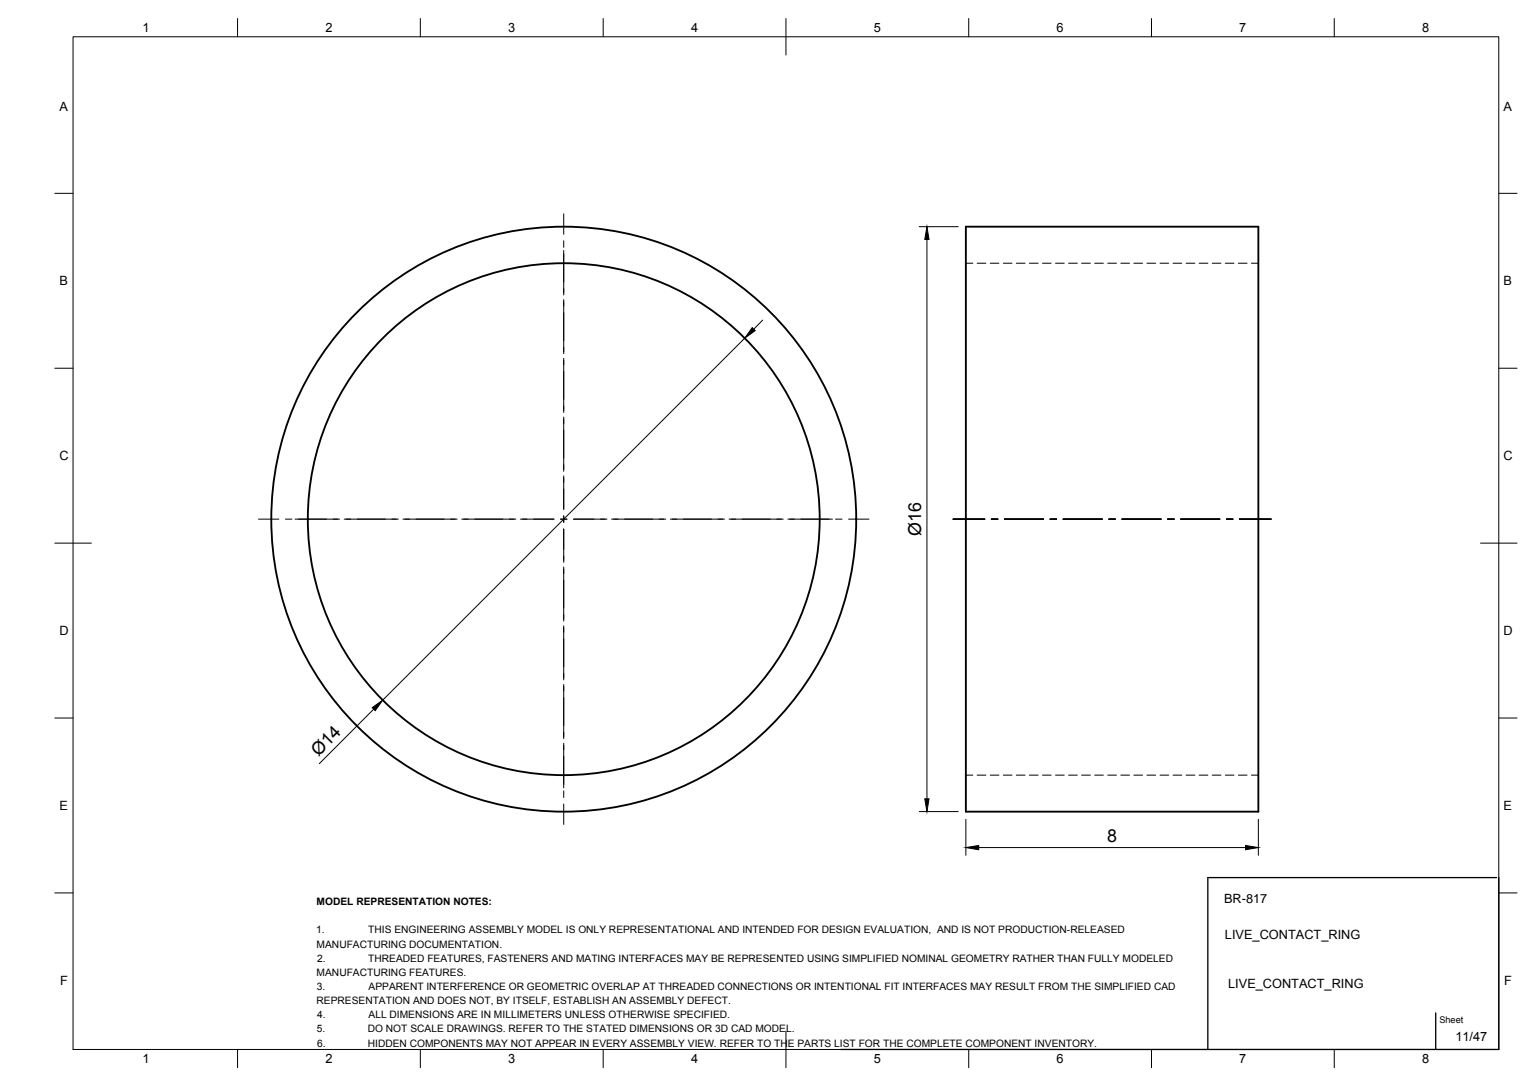
ISO-10303-21;
HEADER;
FILE_DESCRIPTION((''),'2;1');
FILE_NAME('LIVE_CONTACT_RING.step','2026-10-01T22:07:29-07:00',(''),(''),'','','');
FILE_SCHEMA (('AUTOMOTIVE_DESIGN { 1 0 10303 214 3 1 1 }'));
ENDSEC;
DATA;
#10=MECHANICAL_DESIGN_GEOMETRIC_PRESENTATION_REPRESENTATION('',(#547),#15484);
#477=SHAPE_REPRESENTATION_RELATIONSHIP('SRR','None',#15625,#512) ;
#512=ADVANCED_BREP_SHAPE_REPRESENTATION('',(#589),#15449) ;
#547=STYLED_ITEM('',(#15834),#589) ;
#589=MANIFOLD_SOLID_BREP('LIVE_CONTACT_RING',#8256) ;
#654=CYLINDRICAL_SURFACE('',#8850,0.7) ;
#655=CYLINDRICAL_SURFACE('',#8853,0.8) ;
#847=FACE_BOUND('',#2007,.T.) ;
#848=FACE_BOUND('',#2009,.T.) ;
#941=CIRCLE('',#8851,0.7) ;
#942=CIRCLE('',#8852,0.7) ;
#943=CIRCLE('',#8854,0.8) ;
#944=CIRCLE('',#8855,0.8) ;
#1467=FACE_OUTER_BOUND('',#2004,.T.) ;
#1468=FACE_OUTER_BOUND('',#2005,.T.) ;
#1469=FACE_OUTER_BOUND('',#2006,.T.) ;
#1470=FACE_OUTER_BOUND('',#2008,.T.) ;
#2004=EDGE_LOOP('',(#5723,#5724,#5725,#5726)) ;
#2005=EDGE_LOOP('',(#5727,#5728,#5729,#5730)) ;
#2006=EDGE_LOOP('',(#5731)) ;
#2007=EDGE_LOOP('',(#5732)) ;
#2008=EDGE_LOOP('',(#5733)) ;
#2009=EDGE_LOOP('',(#5734)) ;
#2609=LINE('',#13376,#3083) ;
#2610=LINE('',#13382,#3084) ;
#3083=VECTOR('',#10434,0.7) ;
#3084=VECTOR('',#10441,0.8) ;
#3538=VERTEX_POINT('',#13373) ;
#3539=VERTEX_POINT('',#13375) ;
#3540=VERTEX_POINT('',#13379) ;
#3541=VERTEX_POINT('',#13381) ;
#4366=EDGE_CURVE('',#3538,#3538,#941,.T.) ;
#4367=EDGE_CURVE('',#3538,#3539,#2609,.T.) ;
#4368=EDGE_CURVE('',#3539,#3539,#942,.T.) ;
#4369=EDGE_CURVE('',#3540,#3540,#943,.T.) ;
#4370=EDGE_CURVE('',#3540,#3541,#2610,.T.) ;
#4371=EDGE_CURVE('',#3541,#3541,#944,.T.) ;
#5723=ORIENTED_EDGE('',*,*,#4366,.F.) ;
#5724=ORIENTED_EDGE('',*,*,#4367,.T.) ;
#5725=ORIENTED_EDGE('',*,*,#4368,.F.) ;
#5726=ORIENTED_EDGE('',*,*,#4367,.F.) ;
#5727=ORIENTED_EDGE('',*,*,#4369,.F.) ;
#5728=ORIENTED_EDGE('',*,*,#4370,.T.) ;
#5729=ORIENTED_EDGE('',*,*,#4371,.F.) ;
#5730=ORIENTED_EDGE('',*,*,#4370,.F.) ;
#5731=ORIENTED_EDGE('',*,*,#4371,.T.) ;
#5732=ORIENTED_EDGE('',*,*,#4366,.T.) ;
#5733=ORIENTED_EDGE('',*,*,#4369,.T.) ;
#5734=ORIENTED_EDGE('',*,*,#4368,.T.) ;
#7611=PLANE('',#8856) ;
#7612=PLANE('',#8857) ;
#7854=ADVANCED_FACE('',(#1467),#654,.F.) ;
#7855=ADVANCED_FACE('',(#1468),#655,.T.) ;
#7856=ADVANCED_FACE('',(#1469,#847),#7611,.T.) ;
#7857=ADVANCED_FACE('',(#1470,#848),#7612,.T.) ;
#8256=CLOSED_SHELL('',(#7854,#7855,#7856,#7857)) ;
#8849=AXIS2_PLACEMENT_3D('',#13371,#10428,#10429) ;
#8850=AXIS2_PLACEMENT_3D('',#13372,#10430,#10431) ;
#8851=AXIS2_PLACEMENT_3D('',#13374,#10432,#10433) ;
#8852=AXIS2_PLACEMENT_3D('',#13377,#10435,#10436) ;
#8853=AXIS2_PLACEMENT_3D('',#13378,#10437,#10438) ;
#8854=AXIS2_PLACEMENT_3D('',#13380,#10439,#10440) ;
#8855=AXIS2_PLACEMENT_3D('',#13383,#10442,#10443) ;
#8856=AXIS2_PLACEMENT_3D('',#13384,#10444,#10445) ;
#8857=AXIS2_PLACEMENT_3D('',#13385,#10446,#10447) ;
#10428=DIRECTION('axis',(0.,0.,1.)) ;
#10429=DIRECTION('refdir',(1.,0.,0.)) ;
#10430=DIRECTION('center_axis',(0.,0.,1.)) ;
#10431=DIRECTION('ref_axis',(1.,0.,0.)) ;
#10432=DIRECTION('center_axis',(0.,0.,1.)) ;
#10433=DIRECTION('ref_axis',(1.,0.,0.)) ;
#10434=DIRECTION('',(0.,0.,1.)) ;
#10435=DIRECTION('center_axis',(0.,0.,-1.)) ;
#10436=DIRECTION('ref_axis',(1.,0.,0.)) ;
#10437=DIRECTION('center_axis',(0.,0.,1.)) ;
#10438=DIRECTION('ref_axis',(1.,0.,0.)) ;
#10439=DIRECTION('center_axis',(0.,0.,1.)) ;
#10440=DIRECTION('ref_axis',(1.,0.,0.)) ;
#10441=DIRECTION('',(0.,0.,-1.)) ;
#10442=DIRECTION('center_axis',(0.,0.,-1.)) ;
#10443=DIRECTION('ref_axis',(1.,0.,0.)) ;
#10444=DIRECTION('center_axis',(0.,0.,-1.)) ;
#10445=DIRECTION('ref_axis',(-1.,0.,0.)) ;
#10446=DIRECTION('center_axis',(0.,0.,1.)) ;
#10447=DIRECTION('ref_axis',(1.,0.,0.)) ;
#13371=CARTESIAN_POINT('',(0.,0.,0.)) ;
#13372=CARTESIAN_POINT('Origin',(-1.,0.,-0.7)) ;
#13373=CARTESIAN_POINT('',(-1.7,-8.57252759403147E-17,-1.1)) ;
#13374=CARTESIAN_POINT('Origin',(-1.,0.,-1.1)) ;
#13375=CARTESIAN_POINT('',(-1.7,8.57252759403147E-17,-0.3)) ;
#13376=CARTESIAN_POINT('',(-1.7,-8.57252759403147E-17,-0.7)) ;
#13377=CARTESIAN_POINT('Origin',(-1.,0.,-0.3)) ;
#13378=CARTESIAN_POINT('Origin',(-1.,0.,-0.7)) ;
#13379=CARTESIAN_POINT('',(-1.8,-9.79717439317883E-17,-0.3)) ;
#13380=CARTESIAN_POINT('Origin',(-1.,0.,-0.3)) ;
#13381=CARTESIAN_POINT('',(-1.8,-9.79717439317883E-17,-1.1)) ;
#13382=CARTESIAN_POINT('',(-1.8,-9.79717439317883E-17,-0.7)) ;
#13383=CARTESIAN_POINT('Origin',(-1.,0.,-1.1)) ;
#13384=CARTESIAN_POINT('Origin',(-1.,0.,-1.1)) ;
#13385=CARTESIAN_POINT('Origin',(-1.,0.,-0.3)) ;
#15406=UNCERTAINTY_MEASURE_WITH_UNIT(LENGTH_MEASURE(0.001),#15485,
'DISTANCE_ACCURACY_VALUE',
'Maximum model space distance between geometric entities at asserted c
onnectivities') ;
#15441=UNCERTAINTY_MEASURE_WITH_UNIT(LENGTH_MEASURE(0.001),#15485,
'DISTANCE_ACCURACY_VALUE',
'Maximum model space distance between geometric entities at asserted c
onnectivities') ;
#15449=(
GEOMETRIC_REPRESENTATION_CONTEXT(3)
GLOBAL_UNCERTAINTY_ASSIGNED_CONTEXT((#15406))
GLOBAL_UNIT_ASSIGNED_CONTEXT((#15485,#15487,#15488))
REPRESENTATION_CONTEXT('','3D')
) ;
#15484=(
GEOMETRIC_REPRESENTATION_CONTEXT(3)
GLOBAL_UNCERTAINTY_ASSIGNED_CONTEXT((#15441))
GLOBAL_UNIT_ASSIGNED_CONTEXT((#15485,#15487,#15488))
REPRESENTATION_CONTEXT('','3D')
) ;
#15485=(
LENGTH_UNIT()
NAMED_UNIT(*)
SI_UNIT(.CENTI.,.METRE.)
) ;
#15487=(
NAMED_UNIT(*)
PLANE_ANGLE_UNIT()
SI_UNIT($,.RADIAN.)
) ;
#15488=(
NAMED_UNIT(*)
SI_UNIT($,.STERADIAN.)
SOLID_ANGLE_UNIT()
) ;
#15496=SHAPE_DEFINITION_REPRESENTATION(#15540,#15625) ;
#15540=PRODUCT_DEFINITION_SHAPE('',$,#15668) ;
#15625=SHAPE_REPRESENTATION('',(#8849),#15449) ;
#15660=PRODUCT_DEFINITION_CONTEXT('part definition',#15788,'design') ;
#15668=PRODUCT_DEFINITION('LIVE_CONTACT_RING','LIVE_CONTACT_RING',
#15710,#15660) ;
#15710=PRODUCT_DEFINITION_FORMATION('',$,#15797) ;
#15788=APPLICATION_CONTEXT(
'Core Data for Automotive Mechanical Design Process') ;
#15789=PRODUCT_CONTEXT('part definition',#15788,'mechanical') ;
#15797=PRODUCT('LIVE_CONTACT_RING','LIVE_CONTACT_RING',$,(#15789)) ;
#15834=PRESENTATION_STYLE_ASSIGNMENT((#15846)) ;
#15846=SURFACE_STYLE_USAGE(.BOTH.,#15858) ;
#15858=SURFACE_SIDE_STYLE('',(#15870)) ;
#15870=SURFACE_STYLE_FILL_AREA(#15882) ;
#15882=FILL_AREA_STYLE('Brass - Polished',(#15894)) ;
#15894=FILL_AREA_STYLE_COLOUR('Brass - Polished',#15906) ;
#15906=COLOUR_RGB('Brass - Polished', 0.08235294, 0.09019608, 0.10196078) ;
ENDSEC;
END-ISO-10303-21;
